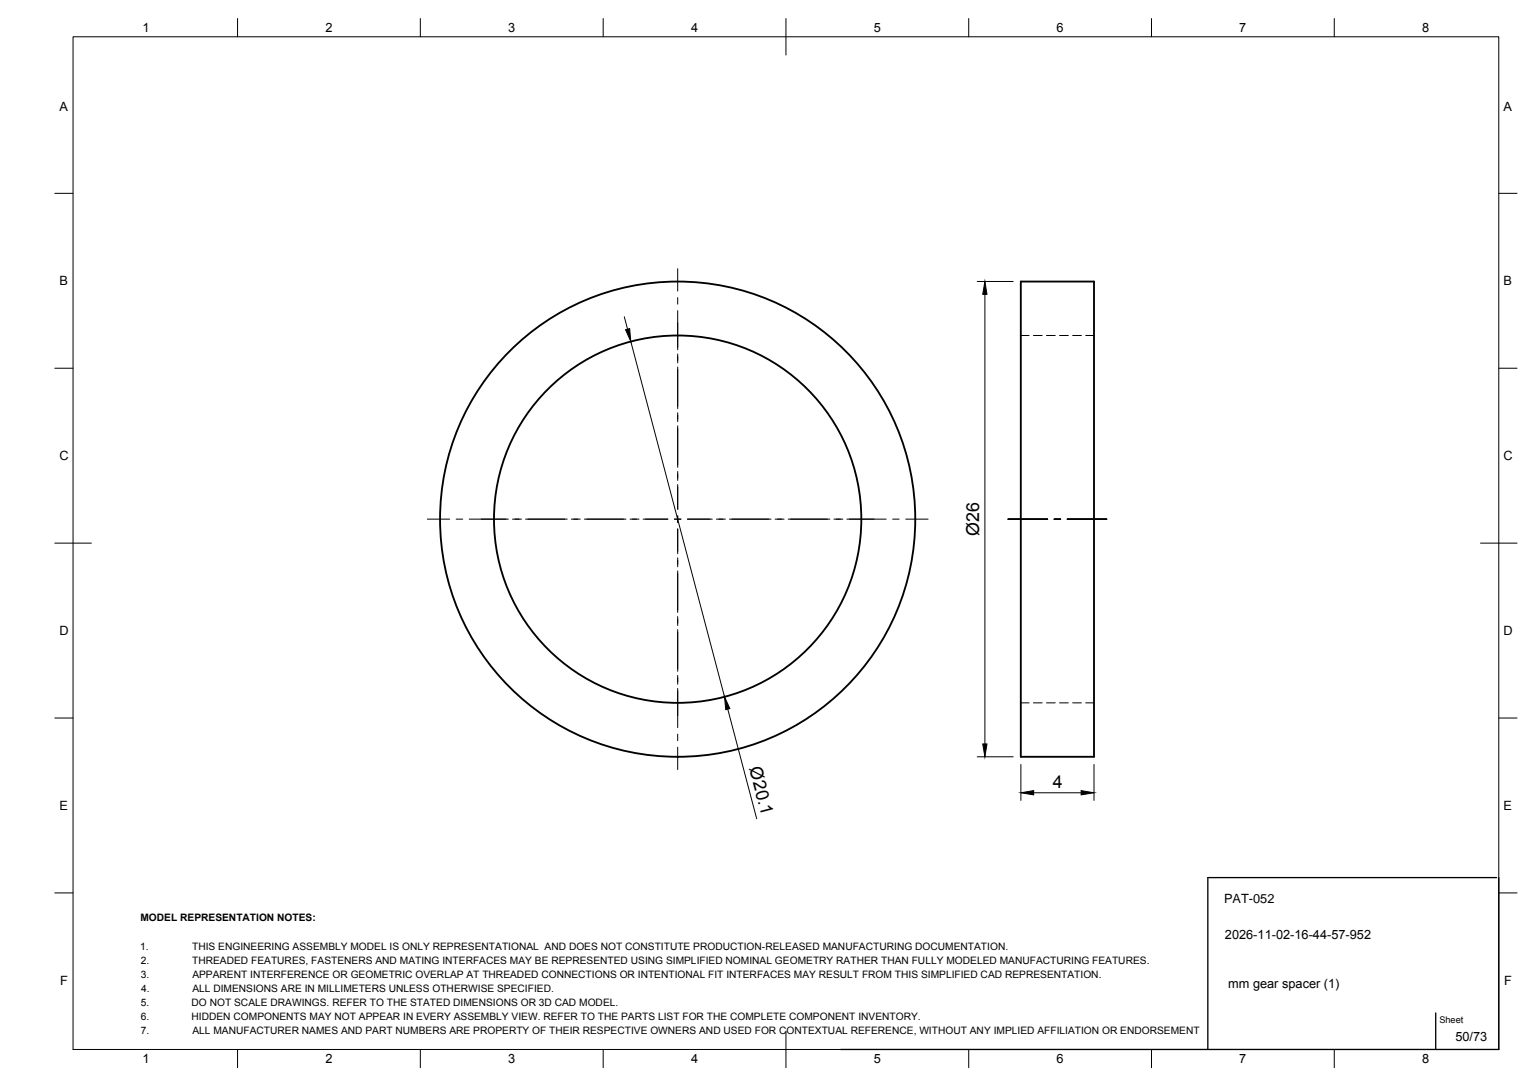
ISO-10303-21;
HEADER;
/* Generated by software containing ST-Developer
 * from STEP Tools, Inc. (www.steptools.com) 
 */

FILE_DESCRIPTION(
/* description */ ('Hand-crank gear train demonstrator'),
/* implementation_level */ '2;1');

FILE_NAME(
/* name */ 'mm gear spacer (1).step',
/* time_stamp */ '2026-10-28T03:22:13-07:00',
/* author */ (''),
/* organization */ (''),
/* preprocessor_version */ 'ST-DEVELOPER v20.2',
/* originating_system */ 'Autodesk Translation Framework v15.17.0.0',
/* authorisation */ '');

FILE_SCHEMA (('AUTOMOTIVE_DESIGN { 1 0 10303 214 3 1 1 }'));
ENDSEC;

DATA;
#10=MECHANICAL_DESIGN_GEOMETRIC_PRESENTATION_REPRESENTATION('',(#1244),#62758);
#1101=SHAPE_REPRESENTATION_RELATIONSHIP('SRR','None',#63077,#1165);
#1165=ADVANCED_BREP_SHAPE_REPRESENTATION('',(#1319),#62731);
#1244=STYLED_ITEM('',(#63476),#1319);
#1319=MANIFOLD_SOLID_BREP('Body1',#16428);
#1576=FACE_BOUND('',#3819,.T.);
#1577=FACE_BOUND('',#3821,.T.);
#1947=PLANE('',#18168);
#1948=PLANE('',#18169);
#2646=FACE_OUTER_BOUND('',#3816,.T.);
#2647=FACE_OUTER_BOUND('',#3817,.T.);
#2648=FACE_OUTER_BOUND('',#3818,.T.);
#2649=FACE_OUTER_BOUND('',#3820,.T.);
#3816=EDGE_LOOP('',(#13071,#13072,#13073,#13074));
#3817=EDGE_LOOP('',(#13075,#13076,#13077,#13078));
#3818=EDGE_LOOP('',(#13079));
#3819=EDGE_LOOP('',(#13080));
#3820=EDGE_LOOP('',(#13081));
#3821=EDGE_LOOP('',(#13082));
#4944=LINE('',#26454,#6076);
#4945=LINE('',#26460,#6077);
#6076=VECTOR('',#21501,1.005);
#6077=VECTOR('',#21508,1.3);
#6974=CIRCLE('',#18163,1.005);
#6975=CIRCLE('',#18164,1.005);
#6976=CIRCLE('',#18166,1.3);
#6977=CIRCLE('',#18167,1.3);
#7971=VERTEX_POINT('',#26451);
#7972=VERTEX_POINT('',#26453);
#7973=VERTEX_POINT('',#26457);
#7974=VERTEX_POINT('',#26459);
#9787=EDGE_CURVE('',#7971,#7971,#6974,.T.);
#9788=EDGE_CURVE('',#7971,#7972,#4944,.T.);
#9789=EDGE_CURVE('',#7972,#7972,#6975,.T.);
#9790=EDGE_CURVE('',#7973,#7973,#6976,.T.);
#9791=EDGE_CURVE('',#7973,#7974,#4945,.T.);
#9792=EDGE_CURVE('',#7974,#7974,#6977,.T.);
#13071=ORIENTED_EDGE('',*,*,#9787,.F.);
#13072=ORIENTED_EDGE('',*,*,#9788,.T.);
#13073=ORIENTED_EDGE('',*,*,#9789,.T.);
#13074=ORIENTED_EDGE('',*,*,#9788,.F.);
#13075=ORIENTED_EDGE('',*,*,#9790,.F.);
#13076=ORIENTED_EDGE('',*,*,#9791,.T.);
#13077=ORIENTED_EDGE('',*,*,#9792,.T.);
#13078=ORIENTED_EDGE('',*,*,#9791,.F.);
#13079=ORIENTED_EDGE('',*,*,#9790,.T.);
#13080=ORIENTED_EDGE('',*,*,#9787,.T.);
#13081=ORIENTED_EDGE('',*,*,#9792,.F.);
#13082=ORIENTED_EDGE('',*,*,#9789,.F.);
#15322=CYLINDRICAL_SURFACE('',#18162,1.005);
#15323=CYLINDRICAL_SURFACE('',#18165,1.3);
#15956=ADVANCED_FACE('',(#2646),#15322,.F.);
#15957=ADVANCED_FACE('',(#2647),#15323,.T.);
#15958=ADVANCED_FACE('',(#2648,#1576),#1947,.T.);
#15959=ADVANCED_FACE('',(#2649,#1577),#1948,.F.);
#16428=CLOSED_SHELL('',(#15956,#15957,#15958,#15959));
#18161=AXIS2_PLACEMENT_3D('',#26449,#21495,#21496);
#18162=AXIS2_PLACEMENT_3D('',#26450,#21497,#21498);
#18163=AXIS2_PLACEMENT_3D('',#26452,#21499,#21500);
#18164=AXIS2_PLACEMENT_3D('',#26455,#21502,#21503);
#18165=AXIS2_PLACEMENT_3D('',#26456,#21504,#21505);
#18166=AXIS2_PLACEMENT_3D('',#26458,#21506,#21507);
#18167=AXIS2_PLACEMENT_3D('',#26461,#21509,#21510);
#18168=AXIS2_PLACEMENT_3D('',#26462,#21511,#21512);
#18169=AXIS2_PLACEMENT_3D('',#26463,#21513,#21514);
#21495=DIRECTION('axis',(0.,0.,1.));
#21496=DIRECTION('refdir',(1.,0.,0.));
#21497=DIRECTION('center_axis',(0.,1.,0.));
#21498=DIRECTION('ref_axis',(1.,0.,0.));
#21499=DIRECTION('center_axis',(0.,-1.,0.));
#21500=DIRECTION('ref_axis',(1.,0.,0.));
#21501=DIRECTION('',(0.,-1.,0.));
#21502=DIRECTION('center_axis',(0.,-1.,0.));
#21503=DIRECTION('ref_axis',(1.,0.,0.));
#21504=DIRECTION('center_axis',(0.,1.,0.));
#21505=DIRECTION('ref_axis',(1.,0.,0.));
#21506=DIRECTION('center_axis',(0.,1.,0.));
#21507=DIRECTION('ref_axis',(1.,0.,0.));
#21508=DIRECTION('',(0.,-1.,0.));
#21509=DIRECTION('center_axis',(0.,1.,0.));
#21510=DIRECTION('ref_axis',(1.,0.,0.));
#21511=DIRECTION('center_axis',(0.,1.,0.));
#21512=DIRECTION('ref_axis',(1.,0.,0.));
#21513=DIRECTION('center_axis',(0.,1.,0.));
#21514=DIRECTION('ref_axis',(1.,0.,0.));
#26449=CARTESIAN_POINT('',(0.,0.,0.));
#26450=CARTESIAN_POINT('Origin',(6.,-0.4,9.));
#26451=CARTESIAN_POINT('',(4.995,0.,9.));
#26452=CARTESIAN_POINT('Origin',(6.,0.,9.));
#26453=CARTESIAN_POINT('',(4.995,-0.4,9.));
#26454=CARTESIAN_POINT('',(4.995,-0.4,9.));
#26455=CARTESIAN_POINT('Origin',(6.,-0.4,9.));
#26456=CARTESIAN_POINT('Origin',(6.,-0.4,9.));
#26457=CARTESIAN_POINT('',(4.7,0.,9.));
#26458=CARTESIAN_POINT('Origin',(6.,0.,9.));
#26459=CARTESIAN_POINT('',(4.7,-0.4,9.));
#26460=CARTESIAN_POINT('',(4.7,-0.4,9.));
#26461=CARTESIAN_POINT('Origin',(6.,-0.4,9.));
#26462=CARTESIAN_POINT('Origin',(6.,0.,9.));
#26463=CARTESIAN_POINT('Origin',(6.,-0.4,9.));
#62657=UNCERTAINTY_MEASURE_WITH_UNIT(LENGTH_MEASURE(0.001),#62759,
'DISTANCE_ACCURACY_VALUE',
'Maximum model space distance between geometric entities at asserted c
onnectivities');
#62684=UNCERTAINTY_MEASURE_WITH_UNIT(LENGTH_MEASURE(0.001),#62759,
'DISTANCE_ACCURACY_VALUE',
'Maximum model space distance between geometric entities at asserted c
onnectivities');
#62731=(
GEOMETRIC_REPRESENTATION_CONTEXT(3)
GLOBAL_UNCERTAINTY_ASSIGNED_CONTEXT((#62657))
GLOBAL_UNIT_ASSIGNED_CONTEXT((#62759,#62761,#62762))
REPRESENTATION_CONTEXT('','3D')
);
#62758=(
GEOMETRIC_REPRESENTATION_CONTEXT(3)
GLOBAL_UNCERTAINTY_ASSIGNED_CONTEXT((#62684))
GLOBAL_UNIT_ASSIGNED_CONTEXT((#62759,#62761,#62762))
REPRESENTATION_CONTEXT('','3D')
);
#62759=(
LENGTH_UNIT()
NAMED_UNIT(*)
SI_UNIT(.CENTI.,.METRE.)
);
#62761=(
NAMED_UNIT(*)
PLANE_ANGLE_UNIT()
SI_UNIT($,.RADIAN.)
);
#62762=(
NAMED_UNIT(*)
SI_UNIT($,.STERADIAN.)
SOLID_ANGLE_UNIT()
);
#62809=SHAPE_DEFINITION_REPRESENTATION(#62892,#63077);
#62892=PRODUCT_DEFINITION_SHAPE('',$,#63151);
#63077=SHAPE_REPRESENTATION('',(#18161),#62731);
#63104=PRODUCT_DEFINITION_CONTEXT('part definition',#63325,'design');
#63151=PRODUCT_DEFINITION('mm gear spacer (1)','mm gear spacer (1)',#63224,
#63104);
#63224=PRODUCT_DEFINITION_FORMATION('',$,#63373);
#63325=APPLICATION_CONTEXT(
'Core Data for Automotive Mechanical Design Process');
#63326=PRODUCT_CONTEXT('part definition',#63325,'mechanical');
#63373=PRODUCT('mm gear spacer (1)','mm gear spacer (1)','mm gear spacer (1)',
(#63326));
#63470=COLOUR_RGB('Off White',0.89,0.88,0.83);
#63471=FILL_AREA_STYLE_COLOUR('',#63470);
#63472=FILL_AREA_STYLE('',(#63471));
#63473=SURFACE_STYLE_FILL_AREA(#63472);
#63474=SURFACE_SIDE_STYLE('',(#63473));
#63475=SURFACE_STYLE_USAGE(.BOTH.,#63474);
#63476=PRESENTATION_STYLE_ASSIGNMENT((#63475));
ENDSEC;
END-ISO-10303-21;
